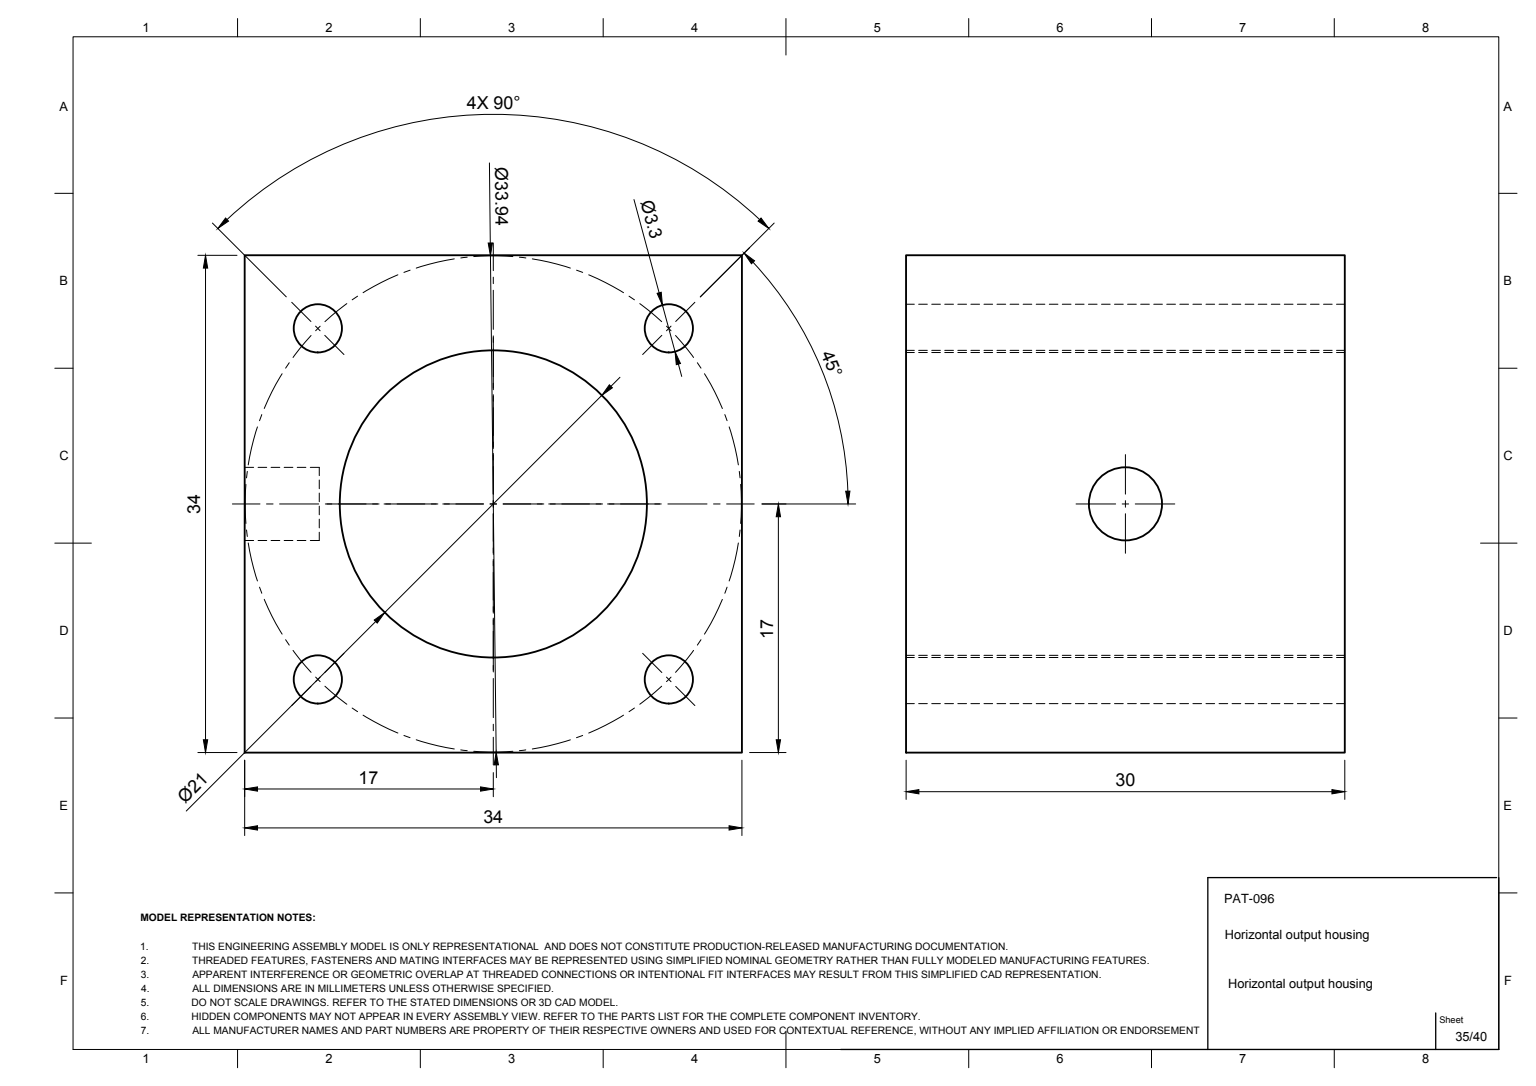
ISO-10303-21;
HEADER;
/* Generated by software containing ST-Developer
 * from STEP Tools, Inc. (www.steptools.com) 
 */

FILE_DESCRIPTION(
/* description */ ('PAT-096'),
/* implementation_level */ '2;1');

FILE_NAME(
/* name */ 'Horizontal output housing.step',
/* time_stamp */ '2026-10-29T17:03:14-07:00',
/* author */ (''),
/* organization */ (''),
/* preprocessor_version */ 'ST-DEVELOPER v20.2',
/* originating_system */ 'Autodesk Translation Framework v15.17.0.0',
/* authorisation */ '');

FILE_SCHEMA (('AUTOMOTIVE_DESIGN { 1 0 10303 214 3 1 1 }'));
ENDSEC;

DATA;
#10=MECHANICAL_DESIGN_GEOMETRIC_PRESENTATION_REPRESENTATION('',(#430),#10650);
#360=SHAPE_REPRESENTATION_RELATIONSHIP('SRR','None',#10824,#391);
#391=ADVANCED_BREP_SHAPE_REPRESENTATION('',(#467),#10642);
#430=STYLED_ITEM('',(#11043),#467);
#467=MANIFOLD_SOLID_BREP('Body1',#5565);
#575=FACE_BOUND('',#1500,.T.);
#576=FACE_BOUND('',#1501,.T.);
#577=FACE_BOUND('',#1502,.T.);
#578=FACE_BOUND('',#1503,.T.);
#579=FACE_BOUND('',#1504,.T.);
#580=FACE_BOUND('',#1507,.T.);
#581=FACE_BOUND('',#1508,.T.);
#582=FACE_BOUND('',#1509,.T.);
#583=FACE_BOUND('',#1510,.T.);
#584=FACE_BOUND('',#1511,.T.);
#585=FACE_BOUND('',#1513,.T.);
#745=PLANE('',#6480);
#746=PLANE('',#6496);
#747=PLANE('',#6497);
#748=PLANE('',#6498);
#749=PLANE('',#6499);
#750=PLANE('',#6500);
#751=PLANE('',#6501);
#1053=FACE_OUTER_BOUND('',#1491,.T.);
#1054=FACE_OUTER_BOUND('',#1492,.T.);
#1055=FACE_OUTER_BOUND('',#1493,.T.);
#1056=FACE_OUTER_BOUND('',#1494,.T.);
#1057=FACE_OUTER_BOUND('',#1495,.T.);
#1058=FACE_OUTER_BOUND('',#1496,.T.);
#1059=FACE_OUTER_BOUND('',#1497,.T.);
#1060=FACE_OUTER_BOUND('',#1498,.T.);
#1061=FACE_OUTER_BOUND('',#1499,.T.);
#1062=FACE_OUTER_BOUND('',#1505,.T.);
#1063=FACE_OUTER_BOUND('',#1506,.T.);
#1064=FACE_OUTER_BOUND('',#1512,.T.);
#1065=FACE_OUTER_BOUND('',#1514,.T.);
#1491=EDGE_LOOP('',(#4779,#4780,#4781,#4782));
#1492=EDGE_LOOP('',(#4783));
#1493=EDGE_LOOP('',(#4784,#4785,#4786,#4787));
#1494=EDGE_LOOP('',(#4788,#4789,#4790,#4791));
#1495=EDGE_LOOP('',(#4792,#4793,#4794,#4795));
#1496=EDGE_LOOP('',(#4796,#4797,#4798,#4799));
#1497=EDGE_LOOP('',(#4800,#4801,#4802,#4803));
#1498=EDGE_LOOP('',(#4804,#4805,#4806,#4807));
#1499=EDGE_LOOP('',(#4808,#4809,#4810,#4811));
#1500=EDGE_LOOP('',(#4812));
#1501=EDGE_LOOP('',(#4813));
#1502=EDGE_LOOP('',(#4814));
#1503=EDGE_LOOP('',(#4815));
#1504=EDGE_LOOP('',(#4816));
#1505=EDGE_LOOP('',(#4817,#4818,#4819,#4820));
#1506=EDGE_LOOP('',(#4821,#4822,#4823,#4824));
#1507=EDGE_LOOP('',(#4825));
#1508=EDGE_LOOP('',(#4826));
#1509=EDGE_LOOP('',(#4827));
#1510=EDGE_LOOP('',(#4828));
#1511=EDGE_LOOP('',(#4829));
#1512=EDGE_LOOP('',(#4830,#4831,#4832,#4833));
#1513=EDGE_LOOP('',(#4834));
#1514=EDGE_LOOP('',(#4835,#4836,#4837,#4838));
#1842=LINE('',#10198,#2171);
#1843=LINE('',#10205,#2172);
#1844=LINE('',#10211,#2173);
#1845=LINE('',#10217,#2174);
#1846=LINE('',#10223,#2175);
#1847=LINE('',#10229,#2176);
#1848=LINE('',#10234,#2177);
#1849=LINE('',#10236,#2178);
#1850=LINE('',#10238,#2179);
#1851=LINE('',#10239,#2180);
#1852=LINE('',#10242,#2181);
#1853=LINE('',#10244,#2182);
#1854=LINE('',#10245,#2183);
#1855=LINE('',#10248,#2184);
#1856=LINE('',#10250,#2185);
#1857=LINE('',#10251,#2186);
#1858=LINE('',#10253,#2187);
#1859=LINE('',#10254,#2188);
#2171=VECTOR('',#8040,0.25);
#2172=VECTOR('',#8049,0.165);
#2173=VECTOR('',#8056,0.165);
#2174=VECTOR('',#8063,0.165);
#2175=VECTOR('',#8070,0.165);
#2176=VECTOR('',#8077,1.05);
#2177=VECTOR('',#8082,1.);
#2178=VECTOR('',#8083,1.);
#2179=VECTOR('',#8084,1.);
#2180=VECTOR('',#8085,1.);
#2181=VECTOR('',#8088,1.);
#2182=VECTOR('',#8089,1.);
#2183=VECTOR('',#8090,1.);
#2184=VECTOR('',#8093,1.);
#2185=VECTOR('',#8094,1.);
#2186=VECTOR('',#8095,1.);
#2187=VECTOR('',#8098,1.);
#2188=VECTOR('',#8099,1.);
#2519=CIRCLE('',#6478,0.25);
#2520=CIRCLE('',#6479,0.25);
#2521=CIRCLE('',#6482,0.165);
#2522=CIRCLE('',#6483,0.165);
#2523=CIRCLE('',#6485,0.165);
#2524=CIRCLE('',#6486,0.165);
#2525=CIRCLE('',#6488,0.165);
#2526=CIRCLE('',#6489,0.165);
#2527=CIRCLE('',#6491,0.165);
#2528=CIRCLE('',#6492,0.165);
#2529=CIRCLE('',#6494,1.05);
#2530=CIRCLE('',#6495,1.05);
#2939=VERTEX_POINT('',#10195);
#2940=VERTEX_POINT('',#10197);
#2941=VERTEX_POINT('',#10202);
#2942=VERTEX_POINT('',#10204);
#2943=VERTEX_POINT('',#10208);
#2944=VERTEX_POINT('',#10210);
#2945=VERTEX_POINT('',#10214);
#2946=VERTEX_POINT('',#10216);
#2947=VERTEX_POINT('',#10220);
#2948=VERTEX_POINT('',#10222);
#2949=VERTEX_POINT('',#10226);
#2950=VERTEX_POINT('',#10228);
#2951=VERTEX_POINT('',#10232);
#2952=VERTEX_POINT('',#10233);
#2953=VERTEX_POINT('',#10235);
#2954=VERTEX_POINT('',#10237);
#2955=VERTEX_POINT('',#10241);
#2956=VERTEX_POINT('',#10243);
#2957=VERTEX_POINT('',#10247);
#2958=VERTEX_POINT('',#10249);
#3568=EDGE_CURVE('',#2939,#2939,#2519,.T.);
#3569=EDGE_CURVE('',#2939,#2940,#1842,.T.);
#3570=EDGE_CURVE('',#2940,#2940,#2520,.T.);
#3571=EDGE_CURVE('',#2941,#2941,#2521,.T.);
#3572=EDGE_CURVE('',#2941,#2942,#1843,.T.);
#3573=EDGE_CURVE('',#2942,#2942,#2522,.T.);
#3574=EDGE_CURVE('',#2943,#2943,#2523,.T.);
#3575=EDGE_CURVE('',#2943,#2944,#1844,.T.);
#3576=EDGE_CURVE('',#2944,#2944,#2524,.T.);
#3577=EDGE_CURVE('',#2945,#2945,#2525,.T.);
#3578=EDGE_CURVE('',#2945,#2946,#1845,.T.);
#3579=EDGE_CURVE('',#2946,#2946,#2526,.T.);
#3580=EDGE_CURVE('',#2947,#2947,#2527,.T.);
#3581=EDGE_CURVE('',#2947,#2948,#1846,.T.);
#3582=EDGE_CURVE('',#2948,#2948,#2528,.T.);
#3583=EDGE_CURVE('',#2949,#2949,#2529,.T.);
#3584=EDGE_CURVE('',#2949,#2950,#1847,.T.);
#3585=EDGE_CURVE('',#2950,#2950,#2530,.T.);
#3586=EDGE_CURVE('',#2951,#2952,#1848,.T.);
#3587=EDGE_CURVE('',#2952,#2953,#1849,.T.);
#3588=EDGE_CURVE('',#2954,#2953,#1850,.T.);
#3589=EDGE_CURVE('',#2951,#2954,#1851,.T.);
#3590=EDGE_CURVE('',#2955,#2951,#1852,.T.);
#3591=EDGE_CURVE('',#2956,#2954,#1853,.T.);
#3592=EDGE_CURVE('',#2955,#2956,#1854,.T.);
#3593=EDGE_CURVE('',#2957,#2955,#1855,.T.);
#3594=EDGE_CURVE('',#2958,#2956,#1856,.T.);
#3595=EDGE_CURVE('',#2957,#2958,#1857,.T.);
#3596=EDGE_CURVE('',#2952,#2957,#1858,.T.);
#3597=EDGE_CURVE('',#2953,#2958,#1859,.T.);
#4779=ORIENTED_EDGE('',*,*,#3568,.F.);
#4780=ORIENTED_EDGE('',*,*,#3569,.T.);
#4781=ORIENTED_EDGE('',*,*,#3570,.F.);
#4782=ORIENTED_EDGE('',*,*,#3569,.F.);
#4783=ORIENTED_EDGE('',*,*,#3568,.T.);
#4784=ORIENTED_EDGE('',*,*,#3571,.F.);
#4785=ORIENTED_EDGE('',*,*,#3572,.T.);
#4786=ORIENTED_EDGE('',*,*,#3573,.F.);
#4787=ORIENTED_EDGE('',*,*,#3572,.F.);
#4788=ORIENTED_EDGE('',*,*,#3574,.F.);
#4789=ORIENTED_EDGE('',*,*,#3575,.T.);
#4790=ORIENTED_EDGE('',*,*,#3576,.F.);
#4791=ORIENTED_EDGE('',*,*,#3575,.F.);
#4792=ORIENTED_EDGE('',*,*,#3577,.F.);
#4793=ORIENTED_EDGE('',*,*,#3578,.T.);
#4794=ORIENTED_EDGE('',*,*,#3579,.F.);
#4795=ORIENTED_EDGE('',*,*,#3578,.F.);
#4796=ORIENTED_EDGE('',*,*,#3580,.F.);
#4797=ORIENTED_EDGE('',*,*,#3581,.T.);
#4798=ORIENTED_EDGE('',*,*,#3582,.F.);
#4799=ORIENTED_EDGE('',*,*,#3581,.F.);
#4800=ORIENTED_EDGE('',*,*,#3583,.F.);
#4801=ORIENTED_EDGE('',*,*,#3584,.T.);
#4802=ORIENTED_EDGE('',*,*,#3585,.F.);
#4803=ORIENTED_EDGE('',*,*,#3584,.F.);
#4804=ORIENTED_EDGE('',*,*,#3586,.T.);
#4805=ORIENTED_EDGE('',*,*,#3587,.T.);
#4806=ORIENTED_EDGE('',*,*,#3588,.F.);
#4807=ORIENTED_EDGE('',*,*,#3589,.F.);
#4808=ORIENTED_EDGE('',*,*,#3590,.T.);
#4809=ORIENTED_EDGE('',*,*,#3589,.T.);
#4810=ORIENTED_EDGE('',*,*,#3591,.F.);
#4811=ORIENTED_EDGE('',*,*,#3592,.F.);
#4812=ORIENTED_EDGE('',*,*,#3585,.T.);
#4813=ORIENTED_EDGE('',*,*,#3582,.T.);
#4814=ORIENTED_EDGE('',*,*,#3579,.T.);
#4815=ORIENTED_EDGE('',*,*,#3576,.T.);
#4816=ORIENTED_EDGE('',*,*,#3573,.T.);
#4817=ORIENTED_EDGE('',*,*,#3593,.T.);
#4818=ORIENTED_EDGE('',*,*,#3592,.T.);
#4819=ORIENTED_EDGE('',*,*,#3594,.F.);
#4820=ORIENTED_EDGE('',*,*,#3595,.F.);
#4821=ORIENTED_EDGE('',*,*,#3596,.T.);
#4822=ORIENTED_EDGE('',*,*,#3595,.T.);
#4823=ORIENTED_EDGE('',*,*,#3597,.F.);
#4824=ORIENTED_EDGE('',*,*,#3587,.F.);
#4825=ORIENTED_EDGE('',*,*,#3583,.T.);
#4826=ORIENTED_EDGE('',*,*,#3580,.T.);
#4827=ORIENTED_EDGE('',*,*,#3577,.T.);
#4828=ORIENTED_EDGE('',*,*,#3574,.T.);
#4829=ORIENTED_EDGE('',*,*,#3571,.T.);
#4830=ORIENTED_EDGE('',*,*,#3597,.T.);
#4831=ORIENTED_EDGE('',*,*,#3594,.T.);
#4832=ORIENTED_EDGE('',*,*,#3591,.T.);
#4833=ORIENTED_EDGE('',*,*,#3588,.T.);
#4834=ORIENTED_EDGE('',*,*,#3570,.T.);
#4835=ORIENTED_EDGE('',*,*,#3596,.F.);
#4836=ORIENTED_EDGE('',*,*,#3586,.F.);
#4837=ORIENTED_EDGE('',*,*,#3590,.F.);
#4838=ORIENTED_EDGE('',*,*,#3593,.F.);
#5170=CYLINDRICAL_SURFACE('',#6477,0.25);
#5171=CYLINDRICAL_SURFACE('',#6481,0.165);
#5172=CYLINDRICAL_SURFACE('',#6484,0.165);
#5173=CYLINDRICAL_SURFACE('',#6487,0.165);
#5174=CYLINDRICAL_SURFACE('',#6490,0.165);
#5175=CYLINDRICAL_SURFACE('',#6493,1.05);
#5458=ADVANCED_FACE('',(#1053),#5170,.F.);
#5459=ADVANCED_FACE('',(#1054),#745,.T.);
#5460=ADVANCED_FACE('',(#1055),#5171,.F.);
#5461=ADVANCED_FACE('',(#1056),#5172,.F.);
#5462=ADVANCED_FACE('',(#1057),#5173,.F.);
#5463=ADVANCED_FACE('',(#1058),#5174,.F.);
#5464=ADVANCED_FACE('',(#1059),#5175,.F.);
#5465=ADVANCED_FACE('',(#1060),#746,.T.);
#5466=ADVANCED_FACE('',(#1061,#575,#576,#577,#578,#579),#747,.T.);
#5467=ADVANCED_FACE('',(#1062),#748,.T.);
#5468=ADVANCED_FACE('',(#1063,#580,#581,#582,#583,#584),#749,.T.);
#5469=ADVANCED_FACE('',(#1064,#585),#750,.T.);
#5470=ADVANCED_FACE('',(#1065),#751,.F.);
#5565=CLOSED_SHELL('',(#5458,#5459,#5460,#5461,#5462,#5463,#5464,#5465,
#5466,#5467,#5468,#5469,#5470));
#6476=AXIS2_PLACEMENT_3D('',#10193,#8034,#8035);
#6477=AXIS2_PLACEMENT_3D('',#10194,#8036,#8037);
#6478=AXIS2_PLACEMENT_3D('',#10196,#8038,#8039);
#6479=AXIS2_PLACEMENT_3D('',#10199,#8041,#8042);
#6480=AXIS2_PLACEMENT_3D('',#10200,#8043,#8044);
#6481=AXIS2_PLACEMENT_3D('',#10201,#8045,#8046);
#6482=AXIS2_PLACEMENT_3D('',#10203,#8047,#8048);
#6483=AXIS2_PLACEMENT_3D('',#10206,#8050,#8051);
#6484=AXIS2_PLACEMENT_3D('',#10207,#8052,#8053);
#6485=AXIS2_PLACEMENT_3D('',#10209,#8054,#8055);
#6486=AXIS2_PLACEMENT_3D('',#10212,#8057,#8058);
#6487=AXIS2_PLACEMENT_3D('',#10213,#8059,#8060);
#6488=AXIS2_PLACEMENT_3D('',#10215,#8061,#8062);
#6489=AXIS2_PLACEMENT_3D('',#10218,#8064,#8065);
#6490=AXIS2_PLACEMENT_3D('',#10219,#8066,#8067);
#6491=AXIS2_PLACEMENT_3D('',#10221,#8068,#8069);
#6492=AXIS2_PLACEMENT_3D('',#10224,#8071,#8072);
#6493=AXIS2_PLACEMENT_3D('',#10225,#8073,#8074);
#6494=AXIS2_PLACEMENT_3D('',#10227,#8075,#8076);
#6495=AXIS2_PLACEMENT_3D('',#10230,#8078,#8079);
#6496=AXIS2_PLACEMENT_3D('',#10231,#8080,#8081);
#6497=AXIS2_PLACEMENT_3D('',#10240,#8086,#8087);
#6498=AXIS2_PLACEMENT_3D('',#10246,#8091,#8092);
#6499=AXIS2_PLACEMENT_3D('',#10252,#8096,#8097);
#6500=AXIS2_PLACEMENT_3D('',#10255,#8100,#8101);
#6501=AXIS2_PLACEMENT_3D('',#10256,#8102,#8103);
#8034=DIRECTION('axis',(0.,0.,1.));
#8035=DIRECTION('refdir',(1.,0.,0.));
#8036=DIRECTION('center_axis',(0.,0.,1.));
#8037=DIRECTION('ref_axis',(1.,0.,0.));
#8038=DIRECTION('center_axis',(0.,0.,1.));
#8039=DIRECTION('ref_axis',(1.,0.,0.));
#8040=DIRECTION('',(0.,0.,1.));
#8041=DIRECTION('center_axis',(0.,0.,-1.));
#8042=DIRECTION('ref_axis',(1.,0.,0.));
#8043=DIRECTION('center_axis',(0.,0.,1.));
#8044=DIRECTION('ref_axis',(1.,0.,0.));
#8045=DIRECTION('center_axis',(1.,0.,0.));
#8046=DIRECTION('ref_axis',(0.,0.,-1.));
#8047=DIRECTION('center_axis',(1.,0.,0.));
#8048=DIRECTION('ref_axis',(0.,0.,-1.));
#8049=DIRECTION('',(1.,0.,0.));
#8050=DIRECTION('center_axis',(-1.,0.,0.));
#8051=DIRECTION('ref_axis',(0.,0.,-1.));
#8052=DIRECTION('center_axis',(1.,0.,0.));
#8053=DIRECTION('ref_axis',(0.,0.,-1.));
#8054=DIRECTION('center_axis',(1.,0.,0.));
#8055=DIRECTION('ref_axis',(0.,0.,-1.));
#8056=DIRECTION('',(1.,0.,0.));
#8057=DIRECTION('center_axis',(-1.,0.,0.));
#8058=DIRECTION('ref_axis',(0.,0.,-1.));
#8059=DIRECTION('center_axis',(1.,0.,0.));
#8060=DIRECTION('ref_axis',(0.,0.,-1.));
#8061=DIRECTION('center_axis',(1.,0.,0.));
#8062=DIRECTION('ref_axis',(0.,0.,-1.));
#8063=DIRECTION('',(1.,0.,0.));
#8064=DIRECTION('center_axis',(-1.,0.,0.));
#8065=DIRECTION('ref_axis',(0.,0.,-1.));
#8066=DIRECTION('center_axis',(1.,0.,0.));
#8067=DIRECTION('ref_axis',(0.,0.,-1.));
#8068=DIRECTION('center_axis',(1.,0.,0.));
#8069=DIRECTION('ref_axis',(0.,0.,-1.));
#8070=DIRECTION('',(1.,0.,0.));
#8071=DIRECTION('center_axis',(-1.,0.,0.));
#8072=DIRECTION('ref_axis',(0.,0.,-1.));
#8073=DIRECTION('center_axis',(1.,0.,0.));
#8074=DIRECTION('ref_axis',(0.,0.,-1.));
#8075=DIRECTION('center_axis',(1.,0.,0.));
#8076=DIRECTION('ref_axis',(0.,0.,-1.));
#8077=DIRECTION('',(1.,0.,0.));
#8078=DIRECTION('center_axis',(-1.,0.,0.));
#8079=DIRECTION('ref_axis',(0.,0.,-1.));
#8080=DIRECTION('center_axis',(0.,1.,0.));
#8081=DIRECTION('ref_axis',(-1.,0.,0.));
#8082=DIRECTION('',(-1.,0.,0.));
#8083=DIRECTION('',(0.,0.,1.));
#8084=DIRECTION('',(-1.,0.,0.));
#8085=DIRECTION('',(0.,0.,1.));
#8086=DIRECTION('center_axis',(1.,0.,0.));
#8087=DIRECTION('ref_axis',(0.,1.,0.));
#8088=DIRECTION('',(0.,1.,0.));
#8089=DIRECTION('',(0.,1.,0.));
#8090=DIRECTION('',(0.,0.,1.));
#8091=DIRECTION('center_axis',(0.,-1.,0.));
#8092=DIRECTION('ref_axis',(1.,0.,0.));
#8093=DIRECTION('',(1.,0.,0.));
#8094=DIRECTION('',(1.,0.,0.));
#8095=DIRECTION('',(0.,0.,1.));
#8096=DIRECTION('center_axis',(-1.,0.,0.));
#8097=DIRECTION('ref_axis',(0.,-1.,0.));
#8098=DIRECTION('',(0.,-1.,0.));
#8099=DIRECTION('',(0.,-1.,0.));
#8100=DIRECTION('center_axis',(0.,0.,1.));
#8101=DIRECTION('ref_axis',(1.,0.,0.));
#8102=DIRECTION('center_axis',(0.,0.,1.));
#8103=DIRECTION('ref_axis',(1.,0.,0.));
#10193=CARTESIAN_POINT('',(0.,0.,0.));
#10194=CARTESIAN_POINT('Origin',(10.,2.,5.19));
#10195=CARTESIAN_POINT('',(9.75,2.,5.19));
#10196=CARTESIAN_POINT('Origin',(10.,2.,5.19));
#10197=CARTESIAN_POINT('',(9.75,2.,5.7));
#10198=CARTESIAN_POINT('',(9.75,2.,5.19));
#10199=CARTESIAN_POINT('Origin',(10.,2.,5.7));
#10200=CARTESIAN_POINT('Origin',(10.,2.,5.19));
#10201=CARTESIAN_POINT('Origin',(8.4,3.2,2.8));
#10202=CARTESIAN_POINT('',(8.5,3.2,2.965));
#10203=CARTESIAN_POINT('Origin',(8.5,3.2,2.8));
#10204=CARTESIAN_POINT('',(11.5,3.2,2.965));
#10205=CARTESIAN_POINT('',(8.4,3.2,2.965));
#10206=CARTESIAN_POINT('Origin',(11.5,3.2,2.8));
#10207=CARTESIAN_POINT('Origin',(8.4,0.8,5.2));
#10208=CARTESIAN_POINT('',(8.5,0.8,5.365));
#10209=CARTESIAN_POINT('Origin',(8.5,0.8,5.2));
#10210=CARTESIAN_POINT('',(11.5,0.8,5.365));
#10211=CARTESIAN_POINT('',(8.4,0.8,5.365));
#10212=CARTESIAN_POINT('Origin',(11.5,0.8,5.2));
#10213=CARTESIAN_POINT('Origin',(8.4,0.8,2.8));
#10214=CARTESIAN_POINT('',(8.5,0.8,2.965));
#10215=CARTESIAN_POINT('Origin',(8.5,0.8,2.8));
#10216=CARTESIAN_POINT('',(11.5,0.8,2.965));
#10217=CARTESIAN_POINT('',(8.4,0.8,2.965));
#10218=CARTESIAN_POINT('Origin',(11.5,0.8,2.8));
#10219=CARTESIAN_POINT('Origin',(8.4,3.2,5.2));
#10220=CARTESIAN_POINT('',(8.5,3.2,5.365));
#10221=CARTESIAN_POINT('Origin',(8.5,3.2,5.2));
#10222=CARTESIAN_POINT('',(11.5,3.2,5.365));
#10223=CARTESIAN_POINT('',(8.4,3.2,5.365));
#10224=CARTESIAN_POINT('Origin',(11.5,3.2,5.2));
#10225=CARTESIAN_POINT('Origin',(8.4,2.,4.));
#10226=CARTESIAN_POINT('',(8.5,2.,5.05));
#10227=CARTESIAN_POINT('Origin',(8.5,2.,4.));
#10228=CARTESIAN_POINT('',(11.5,2.,5.05));
#10229=CARTESIAN_POINT('',(8.4,2.,5.05));
#10230=CARTESIAN_POINT('Origin',(11.5,2.,4.));
#10231=CARTESIAN_POINT('Origin',(11.5,3.7,2.3));
#10232=CARTESIAN_POINT('',(11.5,3.7,2.3));
#10233=CARTESIAN_POINT('',(8.5,3.7,2.3));
#10234=CARTESIAN_POINT('',(11.5,3.7,2.3));
#10235=CARTESIAN_POINT('',(8.5,3.7,5.7));
#10236=CARTESIAN_POINT('',(8.5,3.7,2.3));
#10237=CARTESIAN_POINT('',(11.5,3.7,5.7));
#10238=CARTESIAN_POINT('',(11.5,3.7,5.7));
#10239=CARTESIAN_POINT('',(11.5,3.7,2.3));
#10240=CARTESIAN_POINT('Origin',(11.5,0.3,2.3));
#10241=CARTESIAN_POINT('',(11.5,0.3,2.3));
#10242=CARTESIAN_POINT('',(11.5,0.3,2.3));
#10243=CARTESIAN_POINT('',(11.5,0.3,5.7));
#10244=CARTESIAN_POINT('',(11.5,0.3,5.7));
#10245=CARTESIAN_POINT('',(11.5,0.3,2.3));
#10246=CARTESIAN_POINT('Origin',(8.5,0.3,2.3));
#10247=CARTESIAN_POINT('',(8.5,0.3,2.3));
#10248=CARTESIAN_POINT('',(8.5,0.3,2.3));
#10249=CARTESIAN_POINT('',(8.5,0.3,5.7));
#10250=CARTESIAN_POINT('',(8.5,0.3,5.7));
#10251=CARTESIAN_POINT('',(8.5,0.3,2.3));
#10252=CARTESIAN_POINT('Origin',(8.5,3.7,2.3));
#10253=CARTESIAN_POINT('',(8.5,3.7,2.3));
#10254=CARTESIAN_POINT('',(8.5,3.7,5.7));
#10255=CARTESIAN_POINT('Origin',(10.,2.,5.7));
#10256=CARTESIAN_POINT('Origin',(10.,2.,2.3));
#10603=UNCERTAINTY_MEASURE_WITH_UNIT(LENGTH_MEASURE(0.001),#10651,
'DISTANCE_ACCURACY_VALUE',
'Maximum model space distance between geometric entities at asserted c
onnectivities');
#10611=UNCERTAINTY_MEASURE_WITH_UNIT(LENGTH_MEASURE(0.001),#10651,
'DISTANCE_ACCURACY_VALUE',
'Maximum model space distance between geometric entities at asserted c
onnectivities');
#10642=(
GEOMETRIC_REPRESENTATION_CONTEXT(3)
GLOBAL_UNCERTAINTY_ASSIGNED_CONTEXT((#10603))
GLOBAL_UNIT_ASSIGNED_CONTEXT((#10651,#10653,#10654))
REPRESENTATION_CONTEXT('','3D')
);
#10650=(
GEOMETRIC_REPRESENTATION_CONTEXT(3)
GLOBAL_UNCERTAINTY_ASSIGNED_CONTEXT((#10611))
GLOBAL_UNIT_ASSIGNED_CONTEXT((#10651,#10653,#10654))
REPRESENTATION_CONTEXT('','3D')
);
#10651=(
LENGTH_UNIT()
NAMED_UNIT(*)
SI_UNIT(.CENTI.,.METRE.)
);
#10653=(
NAMED_UNIT(*)
PLANE_ANGLE_UNIT()
SI_UNIT($,.RADIAN.)
);
#10654=(
NAMED_UNIT(*)
SI_UNIT($,.STERADIAN.)
SOLID_ANGLE_UNIT()
);
#10685=SHAPE_DEFINITION_REPRESENTATION(#10731,#10824);
#10731=PRODUCT_DEFINITION_SHAPE('',$,#10863);
#10824=SHAPE_REPRESENTATION('',(#6476),#10642);
#10832=PRODUCT_DEFINITION_CONTEXT('part definition',#10948,'design');
#10863=PRODUCT_DEFINITION('Horizontal output housing',
'Horizontal output housing',#10901,#10832);
#10901=PRODUCT_DEFINITION_FORMATION('',$,#10980);
#10948=APPLICATION_CONTEXT(
'Core Data for Automotive Mechanical Design Process');
#10949=PRODUCT_CONTEXT('part definition',#10948,'mechanical');
#10980=PRODUCT('Horizontal output housing','Horizontal output housing',
'Horizontal output housing',(#10949));
#11037=COLOUR_RGB('Dark Blue',0.08,0.2,0.34);
#11038=FILL_AREA_STYLE_COLOUR('',#11037);
#11039=FILL_AREA_STYLE('',(#11038));
#11040=SURFACE_STYLE_FILL_AREA(#11039);
#11041=SURFACE_SIDE_STYLE('',(#11040));
#11042=SURFACE_STYLE_USAGE(.BOTH.,#11041);
#11043=PRESENTATION_STYLE_ASSIGNMENT((#11042));
ENDSEC;
END-ISO-10303-21;
